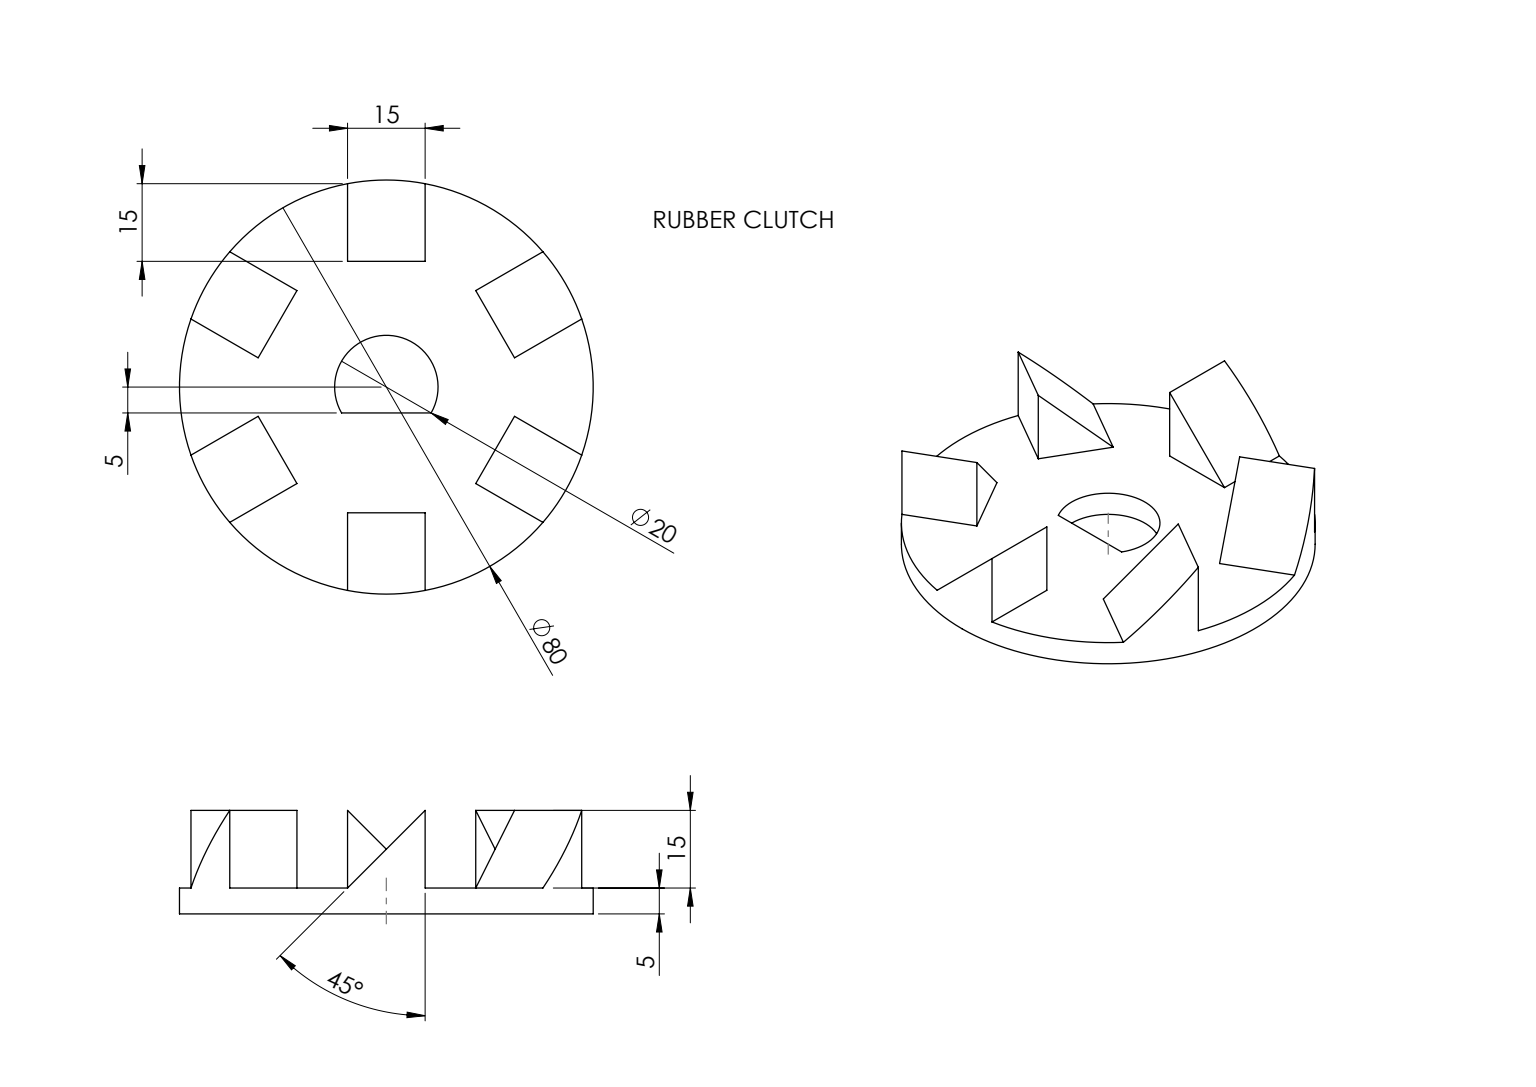
ISO-10303-21;
HEADER;
FILE_DESCRIPTION (('STEP AP214'),
    '1' );
FILE_NAME ('rubber clutch.step',
    '2026-10-09T15:02:13',
    ( '' ),
    ( '' ),
    'SwSTEP 2.0',
    'SolidWorks 2026',
    '' );
FILE_SCHEMA (( 'AUTOMOTIVE_DESIGN' ));
ENDSEC;

DATA;
#35=DIRECTION ( 'NONE',  ( -0.8660254037844327124, 0.000000000000000000, 0.5000000000000102141 ) ) ;
#37=CARTESIAN_POINT ( 'NONE',  ( -24.78626291527390890, 25.00000000000000355, 5.650101528493965297 ) ) ;
#42=CARTESIAN_POINT ( 'NONE',  ( 30.27664397204074476, 25.00000000000000355, 26.14048258526015189 ) ) ;
#92=LINE ( 'NONE', #7754, #12118 ) ;
#146=VECTOR ( 'NONE', #14798, 1000.000000000000000 ) ;
#147=EDGE_CURVE ( 'NONE', #1228, #14186, #15189, .T. ) ;
#226=ORIENTED_EDGE ( 'NONE', *, *, #2314, .T. ) ;
#245=VECTOR ( 'NONE', #10822, 1000.000000000000000 ) ;
#246=ORIENTED_EDGE ( 'NONE', *, *, #11483, .F. ) ;
#251=EDGE_CURVE ( 'NONE', #6737, #5002, #13879, .T. ) ;
#290=LINE ( 'NONE', #6642, #14465 ) ;
#316=SURFACE_SIDE_STYLE ('',( #6586 ) ) ;
#331=VECTOR ( 'NONE', #11777, 1000.000000000000000 ) ;
#372=CARTESIAN_POINT ( 'NONE',  ( -37.77664397204053159, 25.00000000000000355, -13.15010152849376190 ) ) ;
#379=ORIENTED_EDGE ( 'NONE', *, *, #147, .T. ) ;
#392=CARTESIAN_POINT ( 'NONE',  ( -37.77664397204053159, 40.00000000000000711, -13.15010152849376190 ) ) ;
#411=DIRECTION ( 'NONE',  ( -1.000000000000000000, 0.000000000000000000, 2.312964634635742464E-16 ) ) ;
#415=ADVANCED_FACE ( 'NONE', ( #16162 ), #4535, .F. ) ;
#455=EDGE_LOOP ( 'NONE', ( #15919, #7029, #1227 ) ) ;
#484=CARTESIAN_POINT ( 'NONE',  ( 24.78626291527386272, 25.00000000000000355, -5.650101528494135827 ) ) ;
#489=ORIENTED_EDGE ( 'NONE', *, *, #10675, .F. ) ;
#493=DIRECTION ( 'NONE',  ( -0.3535533905932818355, -0.7071067811865463515, -0.6123724356957914727 ) ) ;
#513=ORIENTED_EDGE ( 'NONE', *, *, #11703, .T. ) ;
#524=DIRECTION ( 'NONE',  ( -0.8660254037844399289, 0.000000000000000000, -0.4999999999999976685 ) ) ;
#532=VERTEX_POINT ( 'NONE', #12078 ) ;
#577=EDGE_CURVE ( 'NONE', #11849, #532, #92, .T. ) ;
#585=ORIENTED_EDGE ( 'NONE', *, *, #16374, .T. ) ;
#611=EDGE_LOOP ( 'NONE', ( #10773, #246, #14152, #10214 ) ) ;
#616=DIRECTION ( 'NONE',  ( 0.8660254037844398178, 0.000000000000000000, 0.4999999999999978351 ) ) ;
#641=ORIENTED_EDGE ( 'NONE', *, *, #12919, .T. ) ;
#644=ORIENTED_EDGE ( 'NONE', *, *, #6590, .T. ) ;
#661=STYLED_ITEM ( 'NONE', ( #15532 ), #11759 ) ;
#667=ORIENTED_EDGE ( 'NONE', *, *, #5236, .F. ) ;
#680=VECTOR ( 'NONE', #908, 1000.000000000000000 ) ;
#713=FACE_OUTER_BOUND ( 'NONE', #12733, .T. ) ;
#718=ORIENTED_EDGE ( 'NONE', *, *, #251, .F. ) ;
#758=VERTEX_POINT ( 'NONE', #14387 ) ;
#761=VERTEX_POINT ( 'NONE', #6932 ) ;
#776=MECHANICAL_DESIGN_GEOMETRIC_PRESENTATION_REPRESENTATION('',(#10358),#14324);
#813=LINE ( 'NONE', #10649, #1917 ) ;
#847=FACE_OUTER_BOUND ( 'NONE', #8952, .T. ) ;
#856=AXIS2_PLACEMENT_3D ( 'NONE', #7471, #15025, #3813 ) ;
#858=ORIENTED_EDGE ( 'NONE', *, *, #1166, .T. ) ;
#879=LINE ( 'NONE', #9875, #7578 ) ;
#908=DIRECTION ( 'NONE',  ( 0.5000000000000103251, 0.000000000000000000, 0.8660254037844327124 ) ) ;
#963=EDGE_CURVE ( 'NONE', #14610, #15483, #2393, .T. ) ;
#972=AXIS2_PLACEMENT_3D ( 'NONE', #1664, #10655, #11808 ) ;
#1009=EDGE_CURVE ( 'NONE', #14610, #7079, #9830, .T. ) ;
#1028=ORIENTED_EDGE ( 'NONE', *, *, #8675, .T. ) ;
#1056=CARTESIAN_POINT ( 'NONE',  ( 7.500000000000000000, 40.00000000000000711, 39.29058411375427795 ) ) ;
#1084=CARTESIAN_POINT ( 'NONE',  ( -5.026048470455315886, 27.47395152954465658, 39.76282541253125657 ) ) ;
#1166=EDGE_CURVE ( 'NONE', #13357, #14824, #3055, .T. ) ;
#1181=VERTEX_POINT ( 'NONE', #2335 ) ;
#1202=AXIS2_PLACEMENT_3D ( 'NONE', #5086, #7723, #7477 ) ;
#1210=FACE_OUTER_BOUND ( 'NONE', #4894, .T. ) ;
#1220=DIRECTION ( 'NONE',  ( 0.8660254037844362651, 0.000000000000000000, -0.5000000000000041078 ) ) ;
#1227=ORIENTED_EDGE ( 'NONE', *, *, #9501, .T. ) ;
#1228=VERTEX_POINT ( 'NONE', #484 ) ;
#1231=FACE_OUTER_BOUND ( 'NONE', #5883, .T. ) ;
#1234=( NAMED_UNIT ( * ) SI_UNIT ( $, .STERADIAN. ) SOLID_ANGLE_UNIT ( ) );
#1242=CARTESIAN_POINT ( 'NONE',  ( -36.11321354817274454, 29.97008732934370911, 17.92868204048091840 ) ) ;
#1253=DIRECTION ( 'NONE',  ( 1.000000000000000000, 0.000000000000000000, -2.312964634635742464E-16 ) ) ;
#1282=CIRCLE ( 'NONE', #7664, 40.00000000000000000 ) ;
#1293=DIRECTION ( 'NONE',  ( 0.5000000000000103251, -0.000000000000000000, 0.8660254037844328234 ) ) ;
#1294=CARTESIAN_POINT ( 'NONE',  ( 7.500000000000000000, 25.00000000000000355, 39.29058411375427795 ) ) ;
#1312=COLOUR_RGB ( '', 0.40784314, 0.44705882, 0.49803922) ;
#1317=FACE_OUTER_BOUND ( 'NONE', #13678, .T. ) ;
#1334=EDGE_CURVE ( 'NONE', #13357, #2225, #2828, .T. ) ;
#1374=DIRECTION ( 'NONE',  ( 0.8660254037844327124, 0.000000000000000000, -0.5000000000000102141 ) ) ;
#1386=ORIENTED_EDGE ( 'NONE', *, *, #12039, .T. ) ;
#1399=DIRECTION ( 'NONE',  ( 3.469446951953613696E-16, 0.000000000000000000, 1.000000000000000000 ) ) ;
#1401=AXIS2_PLACEMENT_3D ( 'NONE', #13433, #9616, #10867 ) ;
#1415=ORIENTED_EDGE ( 'NONE', *, *, #13921, .T. ) ;
#1426=CIRCLE ( 'NONE', #12850, 40.00000000000000000 ) ;
#1434=EDGE_CURVE ( 'NONE', #7069, #11084, #1969, .T. ) ;
#1435=UNCERTAINTY_MEASURE_WITH_UNIT (LENGTH_MEASURE( 1.000000000000000082E-05 ), #1651, 'distance_accuracy_value', 'NONE');
#1461=VECTOR ( 'NONE', #16017, 1000.000000000000000 ) ;
#1501=ORIENTED_EDGE ( 'NONE', *, *, #1657, .T. ) ;
#1502=VECTOR ( 'NONE', #1672, 999.9999999999998863 ) ;
#1519=AXIS2_PLACEMENT_3D ( 'NONE', #13845, #1293, #1374 ) ;
#1525=ORIENTED_EDGE ( 'NONE', *, *, #1009, .T. ) ;
#1556=AXIS2_PLACEMENT_3D ( 'NONE', #10146, #14040, #6409 ) ;
#1579=CARTESIAN_POINT ( 'NONE',  ( -17.28626291527383785, 25.00000000000000355, 18.64048258526051427 ) ) ;
#1615=PRODUCT_DEFINITION_SHAPE ( 'NONE', 'NONE',  #14821 ) ;
#1620=ORIENTED_EDGE ( 'NONE', *, *, #4694, .T. ) ;
#1625=EDGE_CURVE ( 'NONE', #3391, #14186, #2782, .T. ) ;
#1651=( LENGTH_UNIT ( ) NAMED_UNIT ( * ) SI_UNIT ( .MILLI., .METRE. ) );
#1657=EDGE_CURVE ( 'NONE', #2087, #5830, #2424, .T. ) ;
#1658=VERTEX_POINT ( 'NONE', #1579 ) ;
#1664=CARTESIAN_POINT ( 'NONE',  ( 0.000000000000000000, 25.00000000000000355, 0.000000000000000000 ) ) ;
#1672=DIRECTION ( 'NONE',  ( -0.8660254037844361541, 0.000000000000000000, 0.5000000000000043299 ) ) ;
#1679=AXIS2_PLACEMENT_3D ( 'NONE', #3745, #10067, #1399 ) ;
#1723=DIRECTION ( 'NONE',  ( 0.000000000000000000, 1.000000000000000000, 0.000000000000000000 ) ) ;
#1812=DIRECTION ( 'NONE',  ( -0.5000000000000041078, 0.000000000000000000, -0.8660254037844363761 ) ) ;
#1824=CARTESIAN_POINT ( 'NONE',  ( -37.77664397204053159, 25.00000000000000355, -13.15010152849376190 ) ) ;
#1843=ORIENTED_EDGE ( 'NONE', *, *, #16366, .F. ) ;
#1848=CARTESIAN_POINT ( 'NONE',  ( -7.500000000000000000, 40.00000000000000711, -39.29058411375427795 ) ) ;
#1851=CARTESIAN_POINT ( 'NONE',  ( 7.500000000000005329, 25.00000000000000355, -24.29058411375428506 ) ) ;
#1861=EDGE_LOOP ( 'NONE', ( #9094, #13992, #14105, #15765 ) ) ;
#1878=ORIENTED_EDGE ( 'NONE', *, *, #3264, .F. ) ;
#1887=DIRECTION ( 'NONE',  ( 0.8660254037844434816, -0.000000000000000000, 0.4999999999999916733 ) ) ;
#1899=FACE_OUTER_BOUND ( 'NONE', #3217, .T. ) ;
#1917=VECTOR ( 'NONE', #11886, 1000.000000000000114 ) ;
#1955=ORIENTED_EDGE ( 'NONE', *, *, #14733, .T. ) ;
#1969=LINE ( 'NONE', #4568, #8682 ) ;
#1971=EDGE_CURVE ( 'NONE', #13357, #6818, #8791, .T. ) ;
#1972=CARTESIAN_POINT ( 'NONE',  ( 0.000000000000000000, 25.00000000000000355, 0.000000000000000000 ) ) ;
#1978=ORIENTED_EDGE ( 'NONE', *, *, #9479, .T. ) ;
#1983=EDGE_LOOP ( 'NONE', ( #585, #8284, #2592, #12178 ) ) ;
#1992=CARTESIAN_POINT ( 'NONE',  ( 37.77664397204061686, 40.00000000000000711, 13.15010152849349900 ) ) ;
#2019=VECTOR ( 'NONE', #16042, 1000.000000000000000 ) ;
#2029=AXIS2_PLACEMENT_3D ( 'NONE', #11411, #2419, #1253 ) ;
#2047=ORIENTED_EDGE ( 'NONE', *, *, #1166, .F. ) ;
#2048=ORIENTED_EDGE ( 'NONE', *, *, #1434, .T. ) ;
#2066=ORIENTED_EDGE ( 'NONE', *, *, #6208, .F. ) ;
#2087=VERTEX_POINT ( 'NONE', #14850 ) ;
#2090=ORIENTED_EDGE ( 'NONE', *, *, #11787, .T. ) ;
#2111=DIRECTION ( 'NONE',  ( 0.000000000000000000, 1.000000000000000000, 0.000000000000000000 ) ) ;
#2135=ADVANCED_FACE ( 'NONE', ( #7219 ), #8534, .F. ) ;
#2158=CARTESIAN_POINT ( 'NONE',  ( 0.000000000000000000, 0.000000000000000000, 0.000000000000000000 ) ) ;
#2172=CARTESIAN_POINT ( 'NONE',  ( -30.27664397204038593, 25.00000000000000355, 26.14048258526057467 ) ) ;
#2173=LINE ( 'NONE', #13488, #9734 ) ;
#2200=VECTOR ( 'NONE', #9579, 1000.000000000000227 ) ;
#2209=CARTESIAN_POINT ( 'NONE',  ( 0.000000000000000000, 20.00000000000000355, 0.000000000000000000 ) ) ;
#2212=LINE ( 'NONE', #15943, #10347 ) ;
#2214=PLANE ( 'NONE',  #15033 ) ;
#2223=EDGE_CURVE ( 'NONE', #6735, #758, #10126, .T. ) ;
#2225=VERTEX_POINT ( 'NONE', #2632 ) ;
#2241=CARTESIAN_POINT ( 'NONE',  ( 37.77664397204061686, 25.00000000000000355, 13.15010152849349900 ) ) ;
#2271=VERTEX_POINT ( 'NONE', #5149 ) ;
#2276=ORIENTED_EDGE ( 'NONE', *, *, #6208, .T. ) ;
#2314=EDGE_CURVE ( 'NONE', #761, #12474, #1282, .T. ) ;
#2329=VECTOR ( 'NONE', #1220, 999.9999999999998863 ) ;
#2335=CARTESIAN_POINT ( 'NONE',  ( 30.27664397204019409, 25.00000000000000355, -26.14048258526078072 ) ) ;
#2340=EDGE_LOOP ( 'NONE', ( #12527, #12705 ) ) ;
#2360=ORIENTED_EDGE ( 'NONE', *, *, #1971, .F. ) ;
#2385=DIRECTION ( 'NONE',  ( 0.000000000000000000, 1.000000000000000000, 0.000000000000000000 ) ) ;
#2393=( BOUNDED_CURVE ( )  B_SPLINE_CURVE ( 3, ( #6008, #10830, #9582, #7252 ),
 .UNSPECIFIED., .F., .F. ) 
 B_SPLINE_CURVE_WITH_KNOTS ( ( 4, 4 ),
 ( 4.523772594209285458, 4.712388980384689674 ),
 .UNSPECIFIED. ) 
 CURVE ( )  GEOMETRIC_REPRESENTATION_ITEM ( )  RATIONAL_B_SPLINE_CURVE ( ( 1.000000000000000000, 0.9970375182503885547, 0.9970375182503885547, 1.000000000000000000 ) ) 
 REPRESENTATION_ITEM ( '' )  );
#2419=DIRECTION ( 'NONE',  ( 2.312964634635742464E-16, -0.000000000000000000, 1.000000000000000000 ) ) ;
#2424=( BOUNDED_CURVE ( )  B_SPLINE_CURVE ( 3, ( #9395, #10571, #4328, #13054 ),
 .UNSPECIFIED., .F., .T. ) 
 B_SPLINE_CURVE_WITH_KNOTS ( ( 4, 4 ),
 ( 4.712388980384689674, 4.901005366560093890 ),
 .UNSPECIFIED. ) 
 CURVE ( )  GEOMETRIC_REPRESENTATION_ITEM ( )  RATIONAL_B_SPLINE_CURVE ( ( 1.000000000000000000, 0.9970375182503885547, 0.9970375182503885547, 1.000000000000000000 ) ) 
 REPRESENTATION_ITEM ( '' )  );
#2436=ORIENTED_EDGE ( 'NONE', *, *, #5698, .F. ) ;
#2439=EDGE_LOOP ( 'NONE', ( #6445, #15228, #12358, #5102, #1525 ) ) ;
#2457=AXIS2_PLACEMENT_3D ( 'NONE', #1972, #13216, #3068 ) ;
#2499=LINE ( 'NONE', #10238, #8412 ) ;
#2516=VERTEX_POINT ( 'NONE', #13471 ) ;
#2517=VECTOR ( 'NONE', #616, 1000.000000000000114 ) ;
#2541=CIRCLE ( 'NONE', #5733, 40.00000000000000000 ) ;
#2561=ADVANCED_FACE ( 'NONE', ( #8981 ), #11314, .F. ) ;
#2571=( LENGTH_UNIT ( ) NAMED_UNIT ( * ) SI_UNIT ( .MILLI., .METRE. ) );
#2592=ORIENTED_EDGE ( 'NONE', *, *, #1625, .F. ) ;
#2632=CARTESIAN_POINT ( 'NONE',  ( -30.27664397204038593, 25.00000000000000355, 26.14048258526057467 ) ) ;
#2657=EDGE_CURVE ( 'NONE', #5002, #2769, #8724, .T. ) ;
#2708=DIRECTION ( 'NONE',  ( -0.3535533905932727872, -0.7071067811865462405, 0.6123724356957966908 ) ) ;
#2724=EDGE_CURVE ( 'NONE', #3391, #5387, #4786, .T. ) ;
#2726=FACE_OUTER_BOUND ( 'NONE', #6080, .T. ) ;
#2747=CARTESIAN_POINT ( 'NONE',  ( -8.660254037844387298, 20.00000000000000355, 5.000000000000000000 ) ) ;
#2765=( BOUNDED_CURVE ( )  B_SPLINE_CURVE ( 3, ( #5034, #10086, #15136, #3763 ),
 .UNSPECIFIED., .F., .F. ) 
 B_SPLINE_CURVE_WITH_KNOTS ( ( 4, 4 ),
 ( 4.523772594209285458, 4.901005366560093002 ),
 .UNSPECIFIED. ) 
 CURVE ( )  GEOMETRIC_REPRESENTATION_ITEM ( )  RATIONAL_B_SPLINE_CURVE ( ( 1.000000000000000000, 0.9881764018959044993, 0.9881764018959044993, 1.000000000000000000 ) ) 
 REPRESENTATION_ITEM ( '' )  );
#2769=VERTEX_POINT ( 'NONE', #15775 ) ;
#2782=LINE ( 'NONE', #11604, #16387 ) ;
#2792=VECTOR ( 'NONE', #7140, 1000.000000000000000 ) ;
#2797=CARTESIAN_POINT ( 'NONE',  ( 24.78626291527397285, 40.00000000000000711, 5.650101528493621572 ) ) ;
#2802=AXIS2_PLACEMENT_3D ( 'NONE', #13583, #2111, #14828 ) ;
#2815=FILL_AREA_STYLE_COLOUR ( '', #1312 ) ;
#2828=LINE ( 'NONE', #14121, #4187 ) ;
#2835=VECTOR ( 'NONE', #5105, 1000.000000000000000 ) ;
#2871=ADVANCED_FACE ( 'NONE', ( #5500 ), #2908, .F. ) ;
#2908=PLANE ( 'NONE',  #12718 ) ;
#2921=CYLINDRICAL_SURFACE ( 'NONE', #972, 40.00000000000000000 ) ;
#2958=DIRECTION ( 'NONE',  ( -0.000000000000000000, -1.000000000000000000, -0.000000000000000000 ) ) ;
#3000=EDGE_CURVE ( 'NONE', #14186, #6058, #2212, .T. ) ;
#3004=LINE ( 'NONE', #9253, #1502 ) ;
#3055=( BOUNDED_CURVE ( )  B_SPLINE_CURVE ( 3, ( #10073, #7734, #1242, #6337 ),
 .UNSPECIFIED., .F., .T. ) 
 B_SPLINE_CURVE_WITH_KNOTS ( ( 4, 4 ),
 ( 4.523772594209285458, 4.901005366560093002 ),
 .UNSPECIFIED. ) 
 CURVE ( )  GEOMETRIC_REPRESENTATION_ITEM ( )  RATIONAL_B_SPLINE_CURVE ( ( 1.000000000000000000, 0.9881764018959044993, 0.9881764018959044993, 1.000000000000000000 ) ) 
 REPRESENTATION_ITEM ( '' )  );
#3068=DIRECTION ( 'NONE',  ( 0.000000000000000000, -0.000000000000000000, 1.000000000000000000 ) ) ;
#3100=ORIENTED_EDGE ( 'NONE', *, *, #6422, .F. ) ;
#3110=EDGE_CURVE ( 'NONE', #9620, #10200, #6470, .T. ) ;
#3135=ORIENTED_EDGE ( 'NONE', *, *, #1334, .F. ) ;
#3140=LINE ( 'NONE', #7970, #6262 ) ;
#3215=ORIENTED_EDGE ( 'NONE', *, *, #6051, .T. ) ;
#3217=EDGE_LOOP ( 'NONE', ( #4738, #5370, #12298, #6596 ) ) ;
#3243=DIRECTION ( 'NONE',  ( 0.3535533905932672916, 0.7071067811865486830, -0.6123724356957968018 ) ) ;
#3264=EDGE_CURVE ( 'NONE', #5374, #758, #10897, .T. ) ;
#3327=DIRECTION ( 'NONE',  ( -0.000000000000000000, -1.000000000000000000, -0.000000000000000000 ) ) ;
#3357=DIRECTION ( 'NONE',  ( 0.8660254037844433705, 0.000000000000000000, 0.4999999999999916178 ) ) ;
#3389=ORIENTED_EDGE ( 'NONE', *, *, #7533, .T. ) ;
#3391=VERTEX_POINT ( 'NONE', #7081 ) ;
#3440=LINE ( 'NONE', #2172, #7521 ) ;
#3445=LINE ( 'NONE', #6028, #16395 ) ;
#3483=DIRECTION ( 'NONE',  ( 0.8660254037844433705, 0.000000000000000000, 0.4999999999999918399 ) ) ;
#3497=EDGE_CURVE ( 'NONE', #14319, #11849, #13789, .T. ) ;
#3540=DIRECTION ( 'NONE',  ( 1.000000000000000000, 0.000000000000000000, 0.000000000000000000 ) ) ;
#3564=CARTESIAN_POINT ( 'NONE',  ( 0.000000000000000000, 25.00000000000000355, 0.000000000000000000 ) ) ;
#3636=MANIFOLD_SOLID_BREP ( 'Cut-Extrude1', #13180 ) ;
#3646=PLANE ( 'NONE',  #1519 ) ;
#3660=ORIENTED_EDGE ( 'NONE', *, *, #7533, .F. ) ;
#3661=ORIENTED_EDGE ( 'NONE', *, *, #9501, .F. ) ;
#3738=ORIENTED_EDGE ( 'NONE', *, *, #9953, .T. ) ;
#3745=CARTESIAN_POINT ( 'NONE',  ( 7.499999999999987566, 40.00000000000000711, -2.602085213965205908E-15 ) ) ;
#3763=CARTESIAN_POINT ( 'NONE',  ( -30.27664397204056712, 25.00000000000000355, -26.14048258526036150 ) ) ;
#3773=DIRECTION ( 'NONE',  ( -0.7071067811865465735, 0.7071067811865484609, 1.635512977795596615E-16 ) ) ;
#3797=CARTESIAN_POINT ( 'NONE',  ( 24.78626291527397285, 25.00000000000000355, 5.650101528493621572 ) ) ;
#3802=CARTESIAN_POINT ( 'NONE',  ( 37.77664397204061686, 40.00000000000000711, 13.15010152849349900 ) ) ;
#3811=AXIS2_PLACEMENT_3D ( 'NONE', #12967, #1812, #6664 ) ;
#3813=DIRECTION ( 'NONE',  ( 0.000000000000000000, 0.000000000000000000, 1.000000000000000000 ) ) ;
#3824=PRESENTATION_STYLE_ASSIGNMENT (( #9228 ) ) ;
#3825=CARTESIAN_POINT ( 'NONE',  ( -7.499999999999998224, 25.00000000000000355, -24.29058411375428150 ) ) ;
#3887=DIRECTION ( 'NONE',  ( 0.000000000000000000, 0.000000000000000000, 1.000000000000000000 ) ) ;
#3907=VECTOR ( 'NONE', #6345, 1000.000000000000000 ) ;
#4028=CARTESIAN_POINT ( 'NONE',  ( -37.77664397204053159, 40.00000000000000711, -13.15010152849376190 ) ) ;
#4067=DIRECTION ( 'NONE',  ( 0.4999999999999978351, 0.000000000000000000, -0.8660254037844399289 ) ) ;
#4069=VECTOR ( 'NONE', #13568, 1000.000000000000114 ) ;
#4077=ORIENTED_EDGE ( 'NONE', *, *, #14561, .T. ) ;
#4084=FACE_OUTER_BOUND ( 'NONE', #12288, .T. ) ;
#4113=ADVANCED_FACE ( 'NONE', ( #1210 ), #10293, .F. ) ;
#4148=PRODUCT ( 'rubber clutch', 'rubber clutch', '', ( #6965 ) ) ;
#4165=FILL_AREA_STYLE ('',( #7895 ) ) ;
#4187=VECTOR ( 'NONE', #10570, 1000.000000000000000 ) ;
#4191=AXIS2_PLACEMENT_3D ( 'NONE', #6061, #13601, #4740 ) ;
#4196=DIRECTION ( 'NONE',  ( -0.8660254037844433705, 0.000000000000000000, -0.4999999999999918399 ) ) ;
#4206=DIRECTION ( 'NONE',  ( -3.469446951953613696E-16, 0.000000000000000000, -1.000000000000000000 ) ) ;
#4231=ORIENTED_EDGE ( 'NONE', *, *, #14339, .T. ) ;
#4236=EDGE_LOOP ( 'NONE', ( #16168, #5571, #11686, #5971 ) ) ;
#4247=( NAMED_UNIT ( * ) PLANE_ANGLE_UNIT ( ) SI_UNIT ( $, .RADIAN. ) );
#4299=LINE ( 'NONE', #14341, #15282 ) ;
#4328=CARTESIAN_POINT ( 'NONE',  ( 5.026048470455315886, 27.47395152954465658, -39.76282541253125657 ) ) ;
#4340=VERTEX_POINT ( 'NONE', #8687 ) ;
#4345=EDGE_CURVE ( 'NONE', #6737, #12652, #6014, .T. ) ;
#4387=EDGE_CURVE ( 'NONE', #12652, #6737, #13752, .T. ) ;
#4418=CARTESIAN_POINT ( 'NONE',  ( 7.499999999999998224, 25.00000000000000355, 24.29058411375428150 ) ) ;
#4535=PLANE ( 'NONE',  #14750 ) ;
#4556=EDGE_LOOP ( 'NONE', ( #15723, #8270, #13295 ) ) ;
#4568=CARTESIAN_POINT ( 'NONE',  ( -24.78626291527393377, 25.00000000000000355, -5.650101528493794767 ) ) ;
#4571=ORIENTED_EDGE ( 'NONE', *, *, #11373, .F. ) ;
#4604=CARTESIAN_POINT ( 'NONE',  ( 0.000000000000000000, 25.00000000000000355, 0.000000000000000000 ) ) ;
#4651=DIRECTION ( 'NONE',  ( -0.000000000000000000, -1.000000000000000000, -0.000000000000000000 ) ) ;
#4694=EDGE_CURVE ( 'NONE', #14169, #2087, #13757, .T. ) ;
#4696=ADVANCED_FACE ( 'NONE', ( #6622 ), #10679, .F. ) ;
#4738=ORIENTED_EDGE ( 'NONE', *, *, #147, .F. ) ;
#4740=DIRECTION ( 'NONE',  ( -1.156482317317871478E-16, 0.000000000000000000, -1.000000000000000000 ) ) ;
#4769=CARTESIAN_POINT ( 'NONE',  ( 30.27664397204019409, 25.00000000000000355, -26.14048258526078072 ) ) ;
#4785=CARTESIAN_POINT ( 'NONE',  ( 3.750000000000036859, 40.00000000000000711, 6.495190528383278483 ) ) ;
#4786=( BOUNDED_CURVE ( )  B_SPLINE_CURVE ( 3, ( #6243, #13954, #12797, #8808 ),
 .UNSPECIFIED., .F., .T. ) 
 B_SPLINE_CURVE_WITH_KNOTS ( ( 4, 4 ),
 ( 4.523772594209285458, 4.901005366560093890 ),
 .UNSPECIFIED. ) 
 CURVE ( )  GEOMETRIC_REPRESENTATION_ITEM ( )  RATIONAL_B_SPLINE_CURVE ( ( 1.000000000000000000, 0.9881764018959044993, 0.9881764018959044993, 1.000000000000000000 ) ) 
 REPRESENTATION_ITEM ( '' )  );
#4793=DIRECTION ( 'NONE',  ( 0.3535533905932685128, -0.7071067811865462405, -0.6123724356957990222 ) ) ;
#4822=LINE ( 'NONE', #12361, #1461 ) ;
#4849=LINE ( 'NONE', #4769, #2200 ) ;
#4856=EDGE_CURVE ( 'NONE', #1228, #5387, #2173, .T. ) ;
#4883=VECTOR ( 'NONE', #6935, 999.9999999999998863 ) ;
#4894=EDGE_LOOP ( 'NONE', ( #8044, #2276, #12130, #7281 ) ) ;
#4897=CARTESIAN_POINT ( 'NONE',  ( -8.660254037844387298, 20.00000000000000355, 5.000000000000000000 ) ) ;
#4922=DIRECTION ( 'NONE',  ( -0.3535533905932715104, 0.7071067811865487940, 0.6123724356957942483 ) ) ;
#5002=VERTEX_POINT ( 'NONE', #9924 ) ;
#5005=ORIENTED_EDGE ( 'NONE', *, *, #6590, .F. ) ;
#5014=PLANE ( 'NONE',  #14232 ) ;
#5028=CARTESIAN_POINT ( 'NONE',  ( 4.898587196589413026E-15, 32.49999999999999289, 40.00000000000000000 ) ) ;
#5034=CARTESIAN_POINT ( 'NONE',  ( -37.77664397204053159, 40.00000000000000711, -13.15010152849376190 ) ) ;
#5053=EDGE_CURVE ( 'NONE', #15026, #14824, #3004, .T. ) ;
#5072=DIRECTION ( 'NONE',  ( -0.8660254037844400399, 0.000000000000000000, -0.4999999999999976685 ) ) ;
#5086=CARTESIAN_POINT ( 'NONE',  ( 0.000000000000000000, 25.00000000000000355, 0.000000000000000000 ) ) ;
#5093=DIRECTION ( 'NONE',  ( -0.8660254037844362651, 0.000000000000000000, 0.5000000000000041078 ) ) ;
#5102=ORIENTED_EDGE ( 'NONE', *, *, #963, .F. ) ;
#5105=DIRECTION ( 'NONE',  ( -0.5000000000000042188, 0.000000000000000000, -0.8660254037844361541 ) ) ;
#5149=CARTESIAN_POINT ( 'NONE',  ( -7.500000000000000000, 25.00000000000000355, 39.29058411375428506 ) ) ;
#5202=ORIENTED_EDGE ( 'NONE', *, *, #12196, .T. ) ;
#5214=EDGE_CURVE ( 'NONE', #2087, #12474, #6854, .T. ) ;
#5236=EDGE_CURVE ( 'NONE', #6058, #1228, #5837, .T. ) ;
#5240=CARTESIAN_POINT ( 'NONE',  ( 7.500000000000000000, 25.00000000000000355, 39.29058411375427795 ) ) ;
#5245=AXIS2_PLACEMENT_3D ( 'NONE', #4604, #9664, #16309 ) ;
#5342=DIRECTION ( 'NONE',  ( -2.312964634635742464E-16, 0.000000000000000000, -1.000000000000000000 ) ) ;
#5353=DIRECTION ( 'NONE',  ( 1.156482317317871478E-16, 0.000000000000000000, 1.000000000000000000 ) ) ;
#5370=ORIENTED_EDGE ( 'NONE', *, *, #4856, .T. ) ;
#5374=VERTEX_POINT ( 'NONE', #2797 ) ;
#5387=VERTEX_POINT ( 'NONE', #7871 ) ;
#5426=EDGE_LOOP ( 'NONE', ( #13925, #3661, #2360, #9220 ) ) ;
#5437=DIRECTION ( 'NONE',  ( -0.4999999999999977796, 0.000000000000000000, 0.8660254037844399289 ) ) ;
#5445=LINE ( 'NONE', #13241, #6201 ) ;
#5481=CIRCLE ( 'NONE', #13419, 40.00000000000000000 ) ;
#5495=VECTOR ( 'NONE', #8882, 1000.000000000000114 ) ;
#5499=DIRECTION ( 'NONE',  ( -0.8660254037844399289, 0.000000000000000000, -0.4999999999999978351 ) ) ;
#5500=FACE_OUTER_BOUND ( 'NONE', #15959, .T. ) ;
#5556=AXIS2_PLACEMENT_3D ( 'NONE', #2209, #7306, #3887 ) ;
#5570=DIRECTION ( 'NONE',  ( 0.8660254037844327124, 0.000000000000000000, -0.5000000000000103251 ) ) ;
#5571=ORIENTED_EDGE ( 'NONE', *, *, #9953, .F. ) ;
#5651=CARTESIAN_POINT ( 'NONE',  ( -24.78626291527393732, 25.00000000000000355, -5.650101528493794767 ) ) ;
#5663=CARTESIAN_POINT ( 'NONE',  ( -3.750000000000069278, 40.00000000000000711, -6.495190528383228745 ) ) ;
#5689=CARTESIAN_POINT ( 'NONE',  ( -5.026048470455357631, 37.52604847045536474, -39.76282541253124947 ) ) ;
#5698=EDGE_CURVE ( 'NONE', #11702, #7069, #12017, .T. ) ;
#5733=AXIS2_PLACEMENT_3D ( 'NONE', #13236, #15644, #15560 ) ;
#5797=PLANE ( 'NONE',  #1401 ) ;
#5830=VERTEX_POINT ( 'NONE', #14744 ) ;
#5837=LINE ( 'NONE', #12306, #680 ) ;
#5843=DIRECTION ( 'NONE',  ( -1.156482317317871478E-16, 0.000000000000000000, -1.000000000000000000 ) ) ;
#5855=DIRECTION ( 'NONE',  ( -0.8660254037844361541, 0.000000000000000000, 0.5000000000000042188 ) ) ;
#5883=EDGE_LOOP ( 'NONE', ( #15156, #12547, #226, #11648, #1501, #3660, #7036, #10674, #10133, #1843, #8414, #15031, #8396 ) ) ;
#5896=DIRECTION ( 'NONE',  ( -0.4999999999999918399, 0.000000000000000000, 0.8660254037844433705 ) ) ;
#5918=LINE ( 'NONE', #10978, #2019 ) ;
#5971=ORIENTED_EDGE ( 'NONE', *, *, #8026, .T. ) ;
#6008=CARTESIAN_POINT ( 'NONE',  ( 7.500000000000000000, 40.00000000000000711, 39.29058411375427795 ) ) ;
#6014=CIRCLE ( 'NONE', #2802, 10.00000000000000000 ) ;
#6015=VECTOR ( 'NONE', #12944, 1000.000000000000000 ) ;
#6024=LINE ( 'NONE', #14976, #4069 ) ;
#6028=CARTESIAN_POINT ( 'NONE',  ( 17.28626291527409720, 25.00000000000000355, 18.64048258526027269 ) ) ;
#6039=ORIENTED_EDGE ( 'NONE', *, *, #4387, .T. ) ;
#6051=EDGE_CURVE ( 'NONE', #11849, #5830, #13327, .T. ) ;
#6058=VERTEX_POINT ( 'NONE', #13088 ) ;
#6061=CARTESIAN_POINT ( 'NONE',  ( -7.500000000000000000, 40.00000000000000711, -39.29058411375427795 ) ) ;
#6072=DIRECTION ( 'NONE',  ( 0.000000000000000000, 1.000000000000000000, 0.000000000000000000 ) ) ;
#6080=EDGE_LOOP ( 'NONE', ( #1978, #718, #10951, #8068 ) ) ;
#6114=DIRECTION ( 'NONE',  ( 0.8660254037844433705, 0.000000000000000000, 0.4999999999999916178 ) ) ;
#6139=CARTESIAN_POINT ( 'NONE',  ( 36.11321354817301454, 35.02991267065631575, 17.92868204048033931 ) ) ;
#6157=ORIENTED_EDGE ( 'NONE', *, *, #5053, .T. ) ;
#6201=VECTOR ( 'NONE', #4196, 1000.000000000000000 ) ;
#6208=EDGE_CURVE ( 'NONE', #11084, #14214, #6873, .T. ) ;
#6215=ORIENTED_EDGE ( 'NONE', *, *, #14733, .F. ) ;
#6239=DIRECTION ( 'NONE',  ( 1.000000000000000000, 0.000000000000000000, -2.312964634635742464E-16 ) ) ;
#6243=CARTESIAN_POINT ( 'NONE',  ( 30.27664397204019409, 40.00000000000000711, -26.14048258526078072 ) ) ;
#6262=VECTOR ( 'NONE', #15444, 1000.000000000000000 ) ;
#6322=ORIENTED_EDGE ( 'NONE', *, *, #12919, .F. ) ;
#6333=CARTESIAN_POINT ( 'NONE',  ( -17.28626291527383785, 40.00000000000000711, 18.64048258526051427 ) ) ;
#6334=EDGE_CURVE ( 'NONE', #10725, #2516, #3445, .T. ) ;
#6337=CARTESIAN_POINT ( 'NONE',  ( -37.77664397204045343, 25.00000000000000355, 13.15010152849403369 ) ) ;
#6345=DIRECTION ( 'NONE',  ( -0.000000000000000000, 1.000000000000000000, -0.000000000000000000 ) ) ;
#6407=DIRECTION ( 'NONE',  ( 0.000000000000000000, 1.000000000000000000, 0.000000000000000000 ) ) ;
#6409=DIRECTION ( 'NONE',  ( 0.000000000000000000, 0.000000000000000000, 1.000000000000000000 ) ) ;
#6410=( NAMED_UNIT ( * ) PLANE_ANGLE_UNIT ( ) SI_UNIT ( $, .RADIAN. ) );
#6422=EDGE_CURVE ( 'NONE', #15026, #6818, #12821, .T. ) ;
#6425=ORIENTED_EDGE ( 'NONE', *, *, #6051, .F. ) ;
#6441=ORIENTED_EDGE ( 'NONE', *, *, #12831, .T. ) ;
#6445=ORIENTED_EDGE ( 'NONE', *, *, #14339, .F. ) ;
#6470=LINE ( 'NONE', #5240, #7943 ) ;
#6586=SURFACE_STYLE_FILL_AREA ( #4165 ) ;
#6590=EDGE_CURVE ( 'NONE', #12474, #761, #2541, .T. ) ;
#6596=ORIENTED_EDGE ( 'NONE', *, *, #1625, .T. ) ;
#6622=FACE_OUTER_BOUND ( 'NONE', #12492, .T. ) ;
#6642=CARTESIAN_POINT ( 'NONE',  ( -24.78626291527393377, 40.00000000000000711, -5.650101528493794767 ) ) ;
#6664=DIRECTION ( 'NONE',  ( -0.8660254037844363761, 0.000000000000000000, 0.5000000000000041078 ) ) ;
#6667=SHAPE_REPRESENTATION_RELATIONSHIP ( 'NONE' , 'NONE' ,  #15095, #11759 ) ;
#6680=ORIENTED_EDGE ( 'NONE', *, *, #16366, .T. ) ;
#6717=LINE ( 'NONE', #15503, #6015 ) ;
#6735=VERTEX_POINT ( 'NONE', #2241 ) ;
#6737=VERTEX_POINT ( 'NONE', #9907 ) ;
#6763=CARTESIAN_POINT ( 'NONE',  ( 0.000000000000000000, 25.00000000000000355, 0.000000000000000000 ) ) ;
#6818=VERTEX_POINT ( 'NONE', #7487 ) ;
#6830=CARTESIAN_POINT ( 'NONE',  ( -7.499999999999998224, 40.00000000000000711, -24.29058411375428150 ) ) ;
#6846=DIRECTION ( 'NONE',  ( 0.8660254037844326014, 0.000000000000000000, -0.5000000000000104361 ) ) ;
#6854=LINE ( 'NONE', #11904, #9997 ) ;
#6873=LINE ( 'NONE', #11924, #14472 ) ;
#6893=DIRECTION ( 'NONE',  ( -0.5000000000000103251, 0.000000000000000000, -0.8660254037844327124 ) ) ;
#6932=CARTESIAN_POINT ( 'NONE',  ( 4.898587196589413026E-15, 20.00000000000000355, 40.00000000000000000 ) ) ;
#6935=DIRECTION ( 'NONE',  ( -0.4999999999999917843, 0.000000000000000000, 0.8660254037844434816 ) ) ;
#6965=PRODUCT_CONTEXT ( 'NONE', #14687, 'mechanical' ) ;
#7002=CARTESIAN_POINT ( 'NONE',  ( -24.78626291527393377, 40.00000000000000711, -5.650101528493794767 ) ) ;
#7029=ORIENTED_EDGE ( 'NONE', *, *, #6422, .T. ) ;
#7036=ORIENTED_EDGE ( 'NONE', *, *, #9462, .F. ) ;
#7044=CARTESIAN_POINT ( 'NONE',  ( 17.28626291527370284, 40.00000000000000711, -18.64048258526063151 ) ) ;
#7069=VERTEX_POINT ( 'NONE', #5651 ) ;
#7079=VERTEX_POINT ( 'NONE', #10568 ) ;
#7081=CARTESIAN_POINT ( 'NONE',  ( 30.27664397204019409, 40.00000000000000711, -26.14048258526078072 ) ) ;
#7118=ORIENTED_EDGE ( 'NONE', *, *, #2223, .T. ) ;
#7140=DIRECTION ( 'NONE',  ( 1.000000000000000000, 0.000000000000000000, 0.000000000000000000 ) ) ;
#7183=PLANE ( 'NONE',  #15199 ) ;
#7219=FACE_OUTER_BOUND ( 'NONE', #611, .T. ) ;
#7221=FACE_OUTER_BOUND ( 'NONE', #4556, .T. ) ;
#7233=ORIENTED_EDGE ( 'NONE', *, *, #9316, .F. ) ;
#7252=CARTESIAN_POINT ( 'NONE',  ( 4.898587196589413026E-15, 32.49999999999999289, 40.00000000000000000 ) ) ;
#7267=DIRECTION ( 'NONE',  ( 0.8660254037844362651, 0.000000000000000000, -0.5000000000000041078 ) ) ;
#7275=VECTOR ( 'NONE', #8643, 1000.000000000000000 ) ;
#7281=ORIENTED_EDGE ( 'NONE', *, *, #15377, .T. ) ;
#7306=DIRECTION ( 'NONE',  ( -0.000000000000000000, 1.000000000000000000, -0.000000000000000000 ) ) ;
#7342=EDGE_LOOP ( 'NONE', ( #9203, #379, #15520 ) ) ;
#7387=CARTESIAN_POINT ( 'NONE',  ( 33.58330087751676984, 29.97008732934371622, 22.31061932476934118 ) ) ;
#7442=( BOUNDED_CURVE ( )  B_SPLINE_CURVE ( 3, ( #3802, #6139, #7387, #42 ),
 .UNSPECIFIED., .F., .F. ) 
 B_SPLINE_CURVE_WITH_KNOTS ( ( 4, 4 ),
 ( 4.523772594209285458, 4.901005366560093002 ),
 .UNSPECIFIED. ) 
 CURVE ( )  GEOMETRIC_REPRESENTATION_ITEM ( )  RATIONAL_B_SPLINE_CURVE ( ( 1.000000000000000000, 0.9881764018959044993, 0.9881764018959044993, 1.000000000000000000 ) ) 
 REPRESENTATION_ITEM ( '' )  );
#7471=CARTESIAN_POINT ( 'NONE',  ( 0.000000000000000000, 25.00000000000000355, 0.000000000000000000 ) ) ;
#7477=DIRECTION ( 'NONE',  ( 0.000000000000000000, 0.000000000000000000, -1.000000000000000000 ) ) ;
#7483=CARTESIAN_POINT ( 'NONE',  ( -7.500000000000005329, 25.00000000000000355, 24.29058411375428506 ) ) ;
#7487=CARTESIAN_POINT ( 'NONE',  ( -17.28626291527383785, 40.00000000000000711, 18.64048258526051427 ) ) ;
#7497=LINE ( 'NONE', #7576, #2835 ) ;
#7521=VECTOR ( 'NONE', #7267, 999.9999999999998863 ) ;
#7533=EDGE_CURVE ( 'NONE', #1181, #5830, #1426, .T. ) ;
#7543=DIRECTION ( 'NONE',  ( 0.000000000000000000, 1.000000000000000000, 0.000000000000000000 ) ) ;
#7576=CARTESIAN_POINT ( 'NONE',  ( -17.28626291527383785, 25.00000000000000355, 18.64048258526051427 ) ) ;
#7578=VECTOR ( 'NONE', #8460, 1000.000000000000000 ) ;
#7623=ORIENTED_EDGE ( 'NONE', *, *, #11598, .T. ) ;
#7664=AXIS2_PLACEMENT_3D ( 'NONE', #13848, #7543, #12613 ) ;
#7723=DIRECTION ( 'NONE',  ( -0.000000000000000000, -1.000000000000000000, -0.000000000000000000 ) ) ;
#7729=PLANE ( 'NONE',  #1679 ) ;
#7734=CARTESIAN_POINT ( 'NONE',  ( -33.58330087751641457, 35.02991267065630154, 22.31061932476987053 ) ) ;
#7754=CARTESIAN_POINT ( 'NONE',  ( -7.499999999999994671, 40.00000000000000711, -24.29058411375428150 ) ) ;
#7801=ORIENTED_EDGE ( 'NONE', *, *, #13221, .T. ) ;
#7804=DIRECTION ( 'NONE',  ( 1.000000000000000000, 0.000000000000000000, 0.000000000000000000 ) ) ;
#7819=ORIENTED_EDGE ( 'NONE', *, *, #13921, .F. ) ;
#7871=CARTESIAN_POINT ( 'NONE',  ( 37.77664397204034685, 25.00000000000000355, -13.15010152849429481 ) ) ;
#7895=FILL_AREA_STYLE_COLOUR ( '', #12889 ) ;
#7943=VECTOR ( 'NONE', #10128, 1000.000000000000000 ) ;
#7960=CARTESIAN_POINT ( 'NONE',  ( -7.500000000000000000, 25.00000000000000355, -39.29058411375427795 ) ) ;
#7964=CARTESIAN_POINT ( 'NONE',  ( 17.28626291527370284, 40.00000000000000711, -18.64048258526062085 ) ) ;
#7970=CARTESIAN_POINT ( 'NONE',  ( 4.898587196589413026E-15, 25.00000000000000355, 40.00000000000000000 ) ) ;
#8026=EDGE_CURVE ( 'NONE', #4340, #11702, #9346, .T. ) ;
#8027=CIRCLE ( 'NONE', #856, 40.00000000000000000 ) ;
#8044=ORIENTED_EDGE ( 'NONE', *, *, #12039, .F. ) ;
#8068=ORIENTED_EDGE ( 'NONE', *, *, #11483, .T. ) ;
#8119=VECTOR ( 'NONE', #3540, 1000.000000000000000 ) ;
#8174=LINE ( 'NONE', #3797, #4883 ) ;
#8182=CARTESIAN_POINT ( 'NONE',  ( 0.000000000000000000, 32.49999999999998579, -40.00000000000000000 ) ) ;
#8206=FACE_OUTER_BOUND ( 'NONE', #7342, .T. ) ;
#8225=FACE_OUTER_BOUND ( 'NONE', #13155, .T. ) ;
#8229=VECTOR ( 'NONE', #6239, 1000.000000000000000 ) ;
#8231=EDGE_LOOP ( 'NONE', ( #6039, #15343 ) ) ;
#8270=ORIENTED_EDGE ( 'NONE', *, *, #10483, .T. ) ;
#8284=ORIENTED_EDGE ( 'NONE', *, *, #3000, .F. ) ;
#8295=CARTESIAN_POINT ( 'NONE',  ( 24.78626291527397285, 40.00000000000000711, 5.650101528493621572 ) ) ;
#8307=ORIENTED_EDGE ( 'NONE', *, *, #1657, .F. ) ;
#8347=VERTEX_POINT ( 'NONE', #12940 ) ;
#8376=LINE ( 'NONE', #16198, #16370 ) ;
#8396=ORIENTED_EDGE ( 'NONE', *, *, #12831, .F. ) ;
#8412=VECTOR ( 'NONE', #5353, 1000.000000000000000 ) ;
#8414=ORIENTED_EDGE ( 'NONE', *, *, #12611, .T. ) ;
#8460=DIRECTION ( 'NONE',  ( -0.000000000000000000, -1.000000000000000000, -0.000000000000000000 ) ) ;
#8471=EDGE_LOOP ( 'NONE', ( #7233, #1028, #7819, #3135, #858, #4571, #15153, #7801, #14636, #16450, #1620, #14149, #644 ) ) ;
#8534=CYLINDRICAL_SURFACE ( 'NONE', #5556, 10.00000000000000000 ) ;
#8536=DIRECTION ( 'NONE',  ( 0.4999999999999916178, 0.000000000000000000, -0.8660254037844433705 ) ) ;
#8560=DIRECTION ( 'NONE',  ( 1.000000000000000000, 0.000000000000000000, 0.000000000000000000 ) ) ;
#8618=DIRECTION ( 'NONE',  ( 0.000000000000000000, 0.000000000000000000, 1.000000000000000000 ) ) ;
#8643=DIRECTION ( 'NONE',  ( -0.000000000000000000, -1.000000000000000000, -0.000000000000000000 ) ) ;
#8674=VECTOR ( 'NONE', #411, 1000.000000000000000 ) ;
#8675=EDGE_CURVE ( 'NONE', #15483, #2271, #13162, .T. ) ;
#8682=VECTOR ( 'NONE', #15780, 1000.000000000000114 ) ;
#8687=CARTESIAN_POINT ( 'NONE',  ( -37.77664397204053159, 40.00000000000000711, -13.15010152849376190 ) ) ;
#8708=DIRECTION ( 'NONE',  ( 3.469446951953613696E-16, 0.000000000000000000, 1.000000000000000000 ) ) ;
#8717=ORIENTED_EDGE ( 'NONE', *, *, #10675, .T. ) ;
#8724=CIRCLE ( 'NONE', #1556, 10.00000000000000000 ) ;
#8783=FACE_OUTER_BOUND ( 'NONE', #1983, .T. ) ;
#8791=LINE ( 'NONE', #13855, #2329 ) ;
#8806=CARTESIAN_POINT ( 'NONE',  ( 0.000000000000000000, 20.00000000000000355, 0.000000000000000000 ) ) ;
#8808=CARTESIAN_POINT ( 'NONE',  ( 37.77664397204034685, 25.00000000000000355, -13.15010152849429481 ) ) ;
#8861=CARTESIAN_POINT ( 'NONE',  ( -7.500000000000000000, 25.00000000000000355, -39.29058411375427795 ) ) ;
#8882=DIRECTION ( 'NONE',  ( -0.3535533905932803922, 0.7071067811865487940, -0.6123724356957891413 ) ) ;
#8884=ORIENTED_EDGE ( 'NONE', *, *, #6334, .F. ) ;
#8888=( NAMED_UNIT ( * ) PLANE_ANGLE_UNIT ( ) SI_UNIT ( $, .RADIAN. ) );
#8952=EDGE_LOOP ( 'NONE', ( #3100, #6157, #2047, #15835 ) ) ;
#8958=CARTESIAN_POINT ( 'NONE',  ( 37.77664397204061686, 25.00000000000000355, 13.15010152849349900 ) ) ;
#8968=ADVANCED_FACE ( 'NONE', ( #2726 ), #15115, .F. ) ;
#8981=FACE_OUTER_BOUND ( 'NONE', #455, .T. ) ;
#9007=AXIS2_PLACEMENT_3D ( 'NONE', #6333, #5093, #13871 ) ;
#9053=ORIENTED_EDGE ( 'NONE', *, *, #3497, .F. ) ;
#9091=VERTEX_POINT ( 'NONE', #10140 ) ;
#9094=ORIENTED_EDGE ( 'NONE', *, *, #10483, .F. ) ;
#9098=DIRECTION ( 'NONE',  ( -0.000000000000000000, -1.000000000000000000, -0.000000000000000000 ) ) ;
#9165=PLANE ( 'NONE',  #14411 ) ;
#9183=CARTESIAN_POINT ( 'NONE',  ( -2.518620260143848100, 35.01862026014384099, -40.00000000000000711 ) ) ;
#9203=ORIENTED_EDGE ( 'NONE', *, *, #5236, .T. ) ;
#9220=ORIENTED_EDGE ( 'NONE', *, *, #1334, .T. ) ;
#9228=SURFACE_STYLE_USAGE ( .BOTH. , #10390 ) ;
#9253=CARTESIAN_POINT ( 'NONE',  ( -24.78626291527390890, 25.00000000000000355, 5.650101528493965297 ) ) ;
#9310=FACE_OUTER_BOUND ( 'NONE', #5426, .T. ) ;
#9316=EDGE_CURVE ( 'NONE', #15483, #761, #3140, .T. ) ;
#9346=LINE ( 'NONE', #4028, #9945 ) ;
#9395=CARTESIAN_POINT ( 'NONE',  ( 0.000000000000000000, 32.49999999999998579, -40.00000000000000000 ) ) ;
#9403=PLANE ( 'NONE',  #13451 ) ;
#9424=AXIS2_PLACEMENT_3D ( 'NONE', #12876, #12546, #7804 ) ;
#9462=EDGE_CURVE ( 'NONE', #3391, #1181, #4822, .T. ) ;
#9479=EDGE_CURVE ( 'NONE', #2769, #5002, #12199, .T. ) ;
#9501=EDGE_CURVE ( 'NONE', #6818, #1658, #879, .T. ) ;
#9547=CARTESIAN_POINT ( 'NONE',  ( 0.000000000000000000, 20.00000000000000355, -40.00000000000000000 ) ) ;
#9575=LINE ( 'NONE', #14619, #11562 ) ;
#9579=DIRECTION ( 'NONE',  ( -0.8660254037844327124, 0.000000000000000000, 0.5000000000000102141 ) ) ;
#9582=CARTESIAN_POINT ( 'NONE',  ( 2.518620260143848100, 35.01862026014384099, 40.00000000000000711 ) ) ;
#9616=DIRECTION ( 'NONE',  ( -1.000000000000000000, 0.000000000000000000, 1.156482317317871478E-16 ) ) ;
#9620=VERTEX_POINT ( 'NONE', #1294 ) ;
#9647=LINE ( 'NONE', #14699, #11835 ) ;
#9664=DIRECTION ( 'NONE',  ( 0.000000000000000000, 1.000000000000000000, 0.000000000000000000 ) ) ;
#9734=VECTOR ( 'NONE', #16157, 1000.000000000000000 ) ;
#9830=LINE ( 'NONE', #12233, #13459 ) ;
#9875=CARTESIAN_POINT ( 'NONE',  ( -17.28626291527383785, 40.00000000000000711, 18.64048258526051427 ) ) ;
#9904=AXIS2_PLACEMENT_3D ( 'NONE', #7044, #5570, #6893 ) ;
#9907=CARTESIAN_POINT ( 'NONE',  ( 8.660254037844387298, 20.00000000000000355, 5.000000000000000000 ) ) ;
#9918=ORIENTED_EDGE ( 'NONE', *, *, #3110, .T. ) ;
#9924=CARTESIAN_POINT ( 'NONE',  ( 8.660254037844387298, 25.00000000000000355, 5.000000000000000000 ) ) ;
#9930=AXIS2_PLACEMENT_3D ( 'NONE', #392, #4067, #5499 ) ;
#9945=VECTOR ( 'NONE', #9098, 1000.000000000000000 ) ;
#9953=EDGE_CURVE ( 'NONE', #8347, #7069, #290, .T. ) ;
#9997=VECTOR ( 'NONE', #14544, 1000.000000000000000 ) ;
#10027=VECTOR ( 'NONE', #4922, 1000.000000000000114 ) ;
#10067=DIRECTION ( 'NONE',  ( 0.7071067811865484609, -0.7071067811865465735, -2.453269466693401579E-16 ) ) ;
#10073=CARTESIAN_POINT ( 'NONE',  ( -30.27664397204038593, 40.00000000000000711, 26.14048258526057467 ) ) ;
#10086=CARTESIAN_POINT ( 'NONE',  ( -36.11321354817288665, 35.02991267065632286, -17.92868204048059155 ) ) ;
#10126=LINE ( 'NONE', #8958, #11643 ) ;
#10128=DIRECTION ( 'NONE',  ( -1.156482317317871478E-16, 0.000000000000000000, -1.000000000000000000 ) ) ;
#10133=ORIENTED_EDGE ( 'NONE', *, *, #12196, .F. ) ;
#10140=CARTESIAN_POINT ( 'NONE',  ( 37.77664397204061686, 40.00000000000000711, 13.15010152849349900 ) ) ;
#10146=CARTESIAN_POINT ( 'NONE',  ( 0.000000000000000000, 25.00000000000000355, 0.000000000000000000 ) ) ;
#10147=( LENGTH_UNIT ( ) NAMED_UNIT ( * ) SI_UNIT ( .MILLI., .METRE. ) );
#10179=ORIENTED_EDGE ( 'NONE', *, *, #11373, .T. ) ;
#10200=VERTEX_POINT ( 'NONE', #14057 ) ;
#10201=ORIENTED_EDGE ( 'NONE', *, *, #15079, .F. ) ;
#10214=ORIENTED_EDGE ( 'NONE', *, *, #251, .T. ) ;
#10238=CARTESIAN_POINT ( 'NONE',  ( -7.500000000000000000, 40.00000000000000711, -39.29058411375427795 ) ) ;
#10273=CIRCLE ( 'NONE', #5245, 40.00000000000000000 ) ;
#10293=PLANE ( 'NONE',  #12094 ) ;
#10301=ORIENTED_EDGE ( 'NONE', *, *, #11787, .F. ) ;
#10314=PLANE ( 'NONE',  #3811 ) ;
#10347=VECTOR ( 'NONE', #4651, 1000.000000000000000 ) ;
#10358=STYLED_ITEM ( 'NONE', ( #3824 ), #3636 ) ;
#10390=SURFACE_SIDE_STYLE ('',( #12792 ) ) ;
#10417=FACE_OUTER_BOUND ( 'NONE', #15056, .T. ) ;
#10433=CARTESIAN_POINT ( 'NONE',  ( -7.499999999999987566, 40.00000000000000711, 2.602085213965205908E-15 ) ) ;
#10479=CARTESIAN_POINT ( 'NONE',  ( -7.500000000000000000, 40.00000000000000711, -39.29058411375427795 ) ) ;
#10483=EDGE_CURVE ( 'NONE', #10725, #5374, #9575, .T. ) ;
#10512=( GEOMETRIC_REPRESENTATION_CONTEXT ( 3 ) GLOBAL_UNCERTAINTY_ASSIGNED_CONTEXT ( ( #14071 ) ) GLOBAL_UNIT_ASSIGNED_CONTEXT ( ( #10147, #6410, #11239 ) ) REPRESENTATION_CONTEXT ( 'NONE', 'WORKASPACE' ) );
#10568=CARTESIAN_POINT ( 'NONE',  ( 7.499999999999998224, 40.00000000000000711, 24.29058411375428150 ) ) ;
#10570=DIRECTION ( 'NONE',  ( -0.000000000000000000, -1.000000000000000000, -0.000000000000000000 ) ) ;
#10571=CARTESIAN_POINT ( 'NONE',  ( 2.518620260143805467, 29.98137973985617677, -40.00000000000000711 ) ) ;
#10578=CARTESIAN_POINT ( 'NONE',  ( 7.500000000000005329, 25.00000000000000355, -24.29058411375428506 ) ) ;
#10584=CARTESIAN_POINT ( 'NONE',  ( 4.898587196589413026E-15, 32.49999999999999289, 40.00000000000000000 ) ) ;
#10636=CARTESIAN_POINT ( 'NONE',  ( 0.000000000000000000, 25.00000000000000355, 0.000000000000000000 ) ) ;
#10649=CARTESIAN_POINT ( 'NONE',  ( 7.499999999999994671, 40.00000000000000711, 24.29058411375428150 ) ) ;
#10655=DIRECTION ( 'NONE',  ( -0.000000000000000000, -1.000000000000000000, -0.000000000000000000 ) ) ;
#10674=ORIENTED_EDGE ( 'NONE', *, *, #2724, .T. ) ;
#10675=EDGE_CURVE ( 'NONE', #532, #14319, #5918, .T. ) ;
#10679=PLANE ( 'NONE',  #11594 ) ;
#10702=VERTEX_POINT ( 'NONE', #7483 ) ;
#10708=DIRECTION ( 'NONE',  ( 0.000000000000000000, 0.000000000000000000, 1.000000000000000000 ) ) ;
#10725=VERTEX_POINT ( 'NONE', #11545 ) ;
#10726=ORIENTED_EDGE ( 'NONE', *, *, #15048, .F. ) ;
#10731=LINE ( 'NONE', #4418, #8674 ) ;
#10773=ORIENTED_EDGE ( 'NONE', *, *, #2657, .T. ) ;
#10780=MECHANICAL_DESIGN_GEOMETRIC_PRESENTATION_REPRESENTATION('',(#661),#13410);
#10822=DIRECTION ( 'NONE',  ( -0.000000000000000000, -1.000000000000000000, -0.000000000000000000 ) ) ;
#10830=CARTESIAN_POINT ( 'NONE',  ( 5.026048470455357631, 37.52604847045536474, 39.76282541253124947 ) ) ;
#10853=ORIENTED_EDGE ( 'NONE', *, *, #11624, .F. ) ;
#10861=ADVANCED_FACE ( 'NONE', ( #16379, #1317 ), #5014, .F. ) ;
#10867=DIRECTION ( 'NONE',  ( 1.156482317317871478E-16, 0.000000000000000000, 1.000000000000000000 ) ) ;
#10897=LINE ( 'NONE', #12396, #245 ) ;
#10951=ORIENTED_EDGE ( 'NONE', *, *, #4387, .F. ) ;
#10978=CARTESIAN_POINT ( 'NONE',  ( -7.499999999999998224, 40.00000000000000711, -24.29058411375428150 ) ) ;
#10989=CARTESIAN_POINT ( 'NONE',  ( 8.660254037844387298, 20.00000000000000355, 5.000000000000000000 ) ) ;
#11054=PRODUCT_DEFINITION_FORMATION_WITH_SPECIFIED_SOURCE ( 'ANY', '', #4148, .NOT_KNOWN. ) ;
#11057=VECTOR ( 'NONE', #14401, 1000.000000000000000 ) ;
#11073=DIRECTION ( 'NONE',  ( 0.000000000000000000, 0.000000000000000000, 1.000000000000000000 ) ) ;
#11084=VERTEX_POINT ( 'NONE', #13994 ) ;
#11193=ORIENTED_EDGE ( 'NONE', *, *, #4856, .F. ) ;
#11239=( NAMED_UNIT ( * ) SI_UNIT ( $, .STERADIAN. ) SOLID_ANGLE_UNIT ( ) );
#11249=EDGE_LOOP ( 'NONE', ( #7118, #1878, #10201, #6680 ) ) ;
#11290=DIRECTION ( 'NONE',  ( -0.8660254037844433705, 0.000000000000000000, -0.4999999999999918399 ) ) ;
#11314=PLANE ( 'NONE',  #9007 ) ;
#11330=CARTESIAN_POINT ( 'NONE',  ( -7.500000000000000000, 25.00000000000000355, 39.29058411375428506 ) ) ;
#11340=CIRCLE ( 'NONE', #12927, 40.00000000000000000 ) ;
#11373=EDGE_CURVE ( 'NONE', #11702, #14824, #10273, .T. ) ;
#11411=CARTESIAN_POINT ( 'NONE',  ( 7.499999999999998224, 40.00000000000000711, 24.29058411375428150 ) ) ;
#11481=PLANE ( 'NONE',  #2029 ) ;
#11483=EDGE_CURVE ( 'NONE', #12652, #2769, #13807, .T. ) ;
#11536=ORIENTED_EDGE ( 'NONE', *, *, #1434, .F. ) ;
#11540=CYLINDRICAL_SURFACE ( 'NONE', #1202, 40.00000000000000000 ) ;
#11545=CARTESIAN_POINT ( 'NONE',  ( 17.28626291527409720, 25.00000000000000355, 18.64048258526027269 ) ) ;
#11559=CARTESIAN_POINT ( 'NONE',  ( -2.518620260143805467, 29.98137973985617677, 40.00000000000000711 ) ) ;
#11562=VECTOR ( 'NONE', #3243, 1000.000000000000114 ) ;
#11594=AXIS2_PLACEMENT_3D ( 'NONE', #10433, #11998, #4206 ) ;
#11598=EDGE_CURVE ( 'NONE', #14169, #532, #2499, .T. ) ;
#11604=CARTESIAN_POINT ( 'NONE',  ( 30.27664397204019409, 40.00000000000000711, -26.14048258526078072 ) ) ;
#11605=ADVANCED_FACE ( 'NONE', ( #4084 ), #11481, .F. ) ;
#11624=EDGE_CURVE ( 'NONE', #1658, #15026, #7497, .T. ) ;
#11643=VECTOR ( 'NONE', #11290, 1000.000000000000000 ) ;
#11648=ORIENTED_EDGE ( 'NONE', *, *, #5214, .F. ) ;
#11686=ORIENTED_EDGE ( 'NONE', *, *, #15377, .F. ) ;
#11702=VERTEX_POINT ( 'NONE', #1824 ) ;
#11703=EDGE_CURVE ( 'NONE', #9620, #2516, #15838, .T. ) ;
#11759=ADVANCED_BREP_SHAPE_REPRESENTATION ( '', ( #3636, #15812 ), #10512 ) ;
#11777=DIRECTION ( 'NONE',  ( 1.156482317317871478E-16, 0.000000000000000000, 1.000000000000000000 ) ) ;
#11779=ADVANCED_FACE ( 'NONE', ( #1899 ), #9403, .F. ) ;
#11787=EDGE_CURVE ( 'NONE', #10200, #10702, #10731, .T. ) ;
#11792=FACE_OUTER_BOUND ( 'NONE', #4236, .T. ) ;
#11808=DIRECTION ( 'NONE',  ( 0.000000000000000000, 0.000000000000000000, -1.000000000000000000 ) ) ;
#11835=VECTOR ( 'NONE', #3327, 1000.000000000000000 ) ;
#11849=VERTEX_POINT ( 'NONE', #10578 ) ;
#11872=ADVANCED_FACE ( 'NONE', ( #14299 ), #2921, .T. ) ;
#11886=DIRECTION ( 'NONE',  ( 0.7071067811865465735, 0.7071067811865484609, -1.635512977795596615E-16 ) ) ;
#11904=CARTESIAN_POINT ( 'NONE',  ( 0.000000000000000000, 25.00000000000000355, -40.00000000000000000 ) ) ;
#11924=CARTESIAN_POINT ( 'NONE',  ( -17.28626291527396930, 25.00000000000000355, -18.64048258526039703 ) ) ;
#11966=ORIENTED_EDGE ( 'NONE', *, *, #2223, .F. ) ;
#11998=DIRECTION ( 'NONE',  ( -0.7071067811865484609, -0.7071067811865465735, 2.453269466693401579E-16 ) ) ;
#12017=LINE ( 'NONE', #372, #2517 ) ;
#12018=SHAPE_DEFINITION_REPRESENTATION ( #1615, #15095 ) ;
#12039=EDGE_CURVE ( 'NONE', #11084, #8347, #14033, .T. ) ;
#12078=CARTESIAN_POINT ( 'NONE',  ( -7.499999999999998224, 40.00000000000000711, -24.29058411375428150 ) ) ;
#12079=ADVANCED_FACE ( 'NONE', ( #1231 ), #11540, .T. ) ;
#12087=ORIENTED_EDGE ( 'NONE', *, *, #577, .T. ) ;
#12094=AXIS2_PLACEMENT_3D ( 'NONE', #16438, #2708, #5072 ) ;
#12118=VECTOR ( 'NONE', #3773, 1000.000000000000114 ) ;
#12124=AXIS2_PLACEMENT_3D ( 'NONE', #6763, #12982, #14450 ) ;
#12130=ORIENTED_EDGE ( 'NONE', *, *, #13221, .F. ) ;
#12178=ORIENTED_EDGE ( 'NONE', *, *, #9462, .T. ) ;
#12182=CARTESIAN_POINT ( 'NONE',  ( -8.660254037844387298, 20.00000000000000355, 5.000000000000000000 ) ) ;
#12196=EDGE_CURVE ( 'NONE', #6735, #5387, #5481, .T. ) ;
#12198=FACE_OUTER_BOUND ( 'NONE', #13521, .T. ) ;
#12199=LINE ( 'NONE', #16192, #2792 ) ;
#12233=CARTESIAN_POINT ( 'NONE',  ( 7.500000000000000000, 40.00000000000000711, 39.29058411375427795 ) ) ;
#12283=CARTESIAN_POINT ( 'NONE',  ( 37.77664397204061686, 40.00000000000000711, 13.15010152849349900 ) ) ;
#12288=EDGE_LOOP ( 'NONE', ( #2090, #4231, #641 ) ) ;
#12298=ORIENTED_EDGE ( 'NONE', *, *, #2724, .F. ) ;
#12306=CARTESIAN_POINT ( 'NONE',  ( 17.28626291527370284, 25.00000000000000355, -18.64048258526063151 ) ) ;
#12358=ORIENTED_EDGE ( 'NONE', *, *, #8675, .F. ) ;
#12361=CARTESIAN_POINT ( 'NONE',  ( 30.27664397204019409, 40.00000000000000711, -26.14048258526078072 ) ) ;
#12396=CARTESIAN_POINT ( 'NONE',  ( 24.78626291527397285, 40.00000000000000711, 5.650101528493621572 ) ) ;
#12416=ADVANCED_FACE ( 'NONE', ( #12198 ), #16107, .F. ) ;
#12474=VERTEX_POINT ( 'NONE', #9547 ) ;
#12492=EDGE_LOOP ( 'NONE', ( #13244, #3215, #8307, #13665, #7623 ) ) ;
#12527=ORIENTED_EDGE ( 'NONE', *, *, #2657, .F. ) ;
#12543=ORIENTED_EDGE ( 'NONE', *, *, #11598, .F. ) ;
#12546=DIRECTION ( 'NONE',  ( -0.000000000000000000, 0.000000000000000000, 1.000000000000000000 ) ) ;
#12547=ORIENTED_EDGE ( 'NONE', *, *, #9316, .T. ) ;
#12611=EDGE_CURVE ( 'NONE', #9091, #2516, #7442, .T. ) ;
#12613=DIRECTION ( 'NONE',  ( 0.000000000000000000, 0.000000000000000000, 1.000000000000000000 ) ) ;
#12623=ADVANCED_FACE ( 'NONE', ( #8783 ), #3646, .F. ) ;
#12652=VERTEX_POINT ( 'NONE', #4897 ) ;
#12705=ORIENTED_EDGE ( 'NONE', *, *, #9479, .F. ) ;
#12716=FILL_AREA_STYLE ('',( #2815 ) ) ;
#12718=AXIS2_PLACEMENT_3D ( 'NONE', #6830, #5342, #14522 ) ;
#12733=EDGE_LOOP ( 'NONE', ( #9918, #6322, #16033, #6441 ) ) ;
#12781=CARTESIAN_POINT ( 'NONE',  ( 0.000000000000000000, 25.00000000000000355, 0.000000000000000000 ) ) ;
#12792=SURFACE_STYLE_FILL_AREA ( #12716 ) ;
#12797=CARTESIAN_POINT ( 'NONE',  ( 36.11321354817260953, 29.97008732934370201, -17.92868204048114222 ) ) ;
#12821=LINE ( 'NONE', #13980, #14765 ) ;
#12831=EDGE_CURVE ( 'NONE', #14610, #9620, #6717, .T. ) ;
#12850=AXIS2_PLACEMENT_3D ( 'NONE', #12781, #6072, #8618 ) ;
#12876=CARTESIAN_POINT ( 'NONE',  ( -8.660254037844387298, 20.00000000000000355, 5.000000000000000000 ) ) ;
#12889=COLOUR_RGB ( '', 0.40784314, 0.44705882, 0.49803922) ;
#12919=EDGE_CURVE ( 'NONE', #7079, #10200, #4299, .T. ) ;
#12927=AXIS2_PLACEMENT_3D ( 'NONE', #3564, #2385, #13689 ) ;
#12940=CARTESIAN_POINT ( 'NONE',  ( -24.78626291527393377, 40.00000000000000711, -5.650101528493794767 ) ) ;
#12944=DIRECTION ( 'NONE',  ( -0.000000000000000000, -1.000000000000000000, -0.000000000000000000 ) ) ;
#12967=CARTESIAN_POINT ( 'NONE',  ( -30.27664397204038593, 40.00000000000000711, 26.14048258526057467 ) ) ;
#12977=CARTESIAN_POINT ( 'NONE',  ( -30.27664397204056712, 25.00000000000000355, -26.14048258526036150 ) ) ;
#12982=DIRECTION ( 'NONE',  ( 0.000000000000000000, 1.000000000000000000, 0.000000000000000000 ) ) ;
#13050=SURFACE_STYLE_USAGE ( .BOTH. , #316 ) ;
#13054=CARTESIAN_POINT ( 'NONE',  ( 7.500000000000000000, 25.00000000000000355, -39.29058411375427795 ) ) ;
#13056=ORIENTED_EDGE ( 'NONE', *, *, #5053, .F. ) ;
#13088=CARTESIAN_POINT ( 'NONE',  ( 17.28626291527369929, 25.00000000000000355, -18.64048258526063151 ) ) ;
#13122=PLANE ( 'NONE',  #9930 ) ;
#13155=EDGE_LOOP ( 'NONE', ( #11193, #667, #16325, #3389, #6425, #9053, #6215, #4077, #2066, #11536, #2436, #10179, #13056, #10853, #15654, #1415, #15112, #10301, #13319, #513, #8884, #10726, #11966, #5202 ) ) ;
#13162=( BOUNDED_CURVE ( )  B_SPLINE_CURVE ( 3, ( #5028, #11559, #1084, #11330 ),
 .UNSPECIFIED., .F., .F. ) 
 B_SPLINE_CURVE_WITH_KNOTS ( ( 4, 4 ),
 ( 4.712388980384689674, 4.901005366560093890 ),
 .UNSPECIFIED. ) 
 CURVE ( )  GEOMETRIC_REPRESENTATION_ITEM ( )  RATIONAL_B_SPLINE_CURVE ( ( 1.000000000000000000, 0.9970375182503885547, 0.9970375182503885547, 1.000000000000000000 ) ) 
 REPRESENTATION_ITEM ( '' )  );
#13180=CLOSED_SHELL ( 'NONE', ( #12079, #11872, #14357, #10861, #12416, #2871, #4696, #16117, #16345, #16071, #2561, #14865, #11605, #13973, #16172, #12623, #14820, #4113, #15286, #15987, #415, #11779, #2135, #8968 ) ) ;
#13200=ORIENTED_EDGE ( 'NONE', *, *, #3497, .T. ) ;
#13216=DIRECTION ( 'NONE',  ( 0.000000000000000000, 1.000000000000000000, 0.000000000000000000 ) ) ;
#13221=EDGE_CURVE ( 'NONE', #4340, #14214, #2765, .T. ) ;
#13236=CARTESIAN_POINT ( 'NONE',  ( 0.000000000000000000, 20.00000000000000355, 0.000000000000000000 ) ) ;
#13241=CARTESIAN_POINT ( 'NONE',  ( 37.77664397204061686, 40.00000000000000711, 13.15010152849349900 ) ) ;
#13244=ORIENTED_EDGE ( 'NONE', *, *, #577, .F. ) ;
#13274=CARTESIAN_POINT ( 'NONE',  ( -37.77664397204045343, 25.00000000000000355, 13.15010152849403369 ) ) ;
#13295=ORIENTED_EDGE ( 'NONE', *, *, #3264, .T. ) ;
#13319=ORIENTED_EDGE ( 'NONE', *, *, #3110, .F. ) ;
#13327=LINE ( 'NONE', #1851, #11057 ) ;
#13357=VERTEX_POINT ( 'NONE', #15711 ) ;
#13363=PLANE ( 'NONE',  #15208 ) ;
#13410=( GEOMETRIC_REPRESENTATION_CONTEXT ( 3 ) GLOBAL_UNCERTAINTY_ASSIGNED_CONTEXT ( ( #1435 ) ) GLOBAL_UNIT_ASSIGNED_CONTEXT ( ( #1651, #4247, #15622 ) ) REPRESENTATION_CONTEXT ( 'NONE', 'WORKASPACE' ) );
#13419=AXIS2_PLACEMENT_3D ( 'NONE', #10636, #1723, #10708 ) ;
#13433=CARTESIAN_POINT ( 'NONE',  ( 7.500000000000000000, 40.00000000000000711, 39.29058411375427795 ) ) ;
#13451=AXIS2_PLACEMENT_3D ( 'NONE', #5663, #493, #6846 ) ;
#13452=FACE_OUTER_BOUND ( 'NONE', #11249, .T. ) ;
#13459=VECTOR ( 'NONE', #5843, 1000.000000000000000 ) ;
#13471=CARTESIAN_POINT ( 'NONE',  ( 30.27664397204074476, 25.00000000000000355, 26.14048258526015189 ) ) ;
#13488=CARTESIAN_POINT ( 'NONE',  ( 24.78626291527386272, 25.00000000000000355, -5.650101528494135827 ) ) ;
#13521=EDGE_LOOP ( 'NONE', ( #1955, #489, #12543, #15574 ) ) ;
#13561=EDGE_CURVE ( 'NONE', #14169, #15028, #9647, .T. ) ;
#13568=DIRECTION ( 'NONE',  ( 0.8660254037844398178, 0.000000000000000000, 0.4999999999999978351 ) ) ;
#13583=CARTESIAN_POINT ( 'NONE',  ( 0.000000000000000000, 20.00000000000000355, 0.000000000000000000 ) ) ;
#13601=DIRECTION ( 'NONE',  ( 1.000000000000000000, 0.000000000000000000, -1.156482317317871478E-16 ) ) ;
#13655=CARTESIAN_POINT ( 'NONE',  ( 3.749999999999932943, 40.00000000000000711, -6.495190528383318451 ) ) ;
#13665=ORIENTED_EDGE ( 'NONE', *, *, #4694, .F. ) ;
#13678=EDGE_LOOP ( 'NONE', ( #5005, #14371 ) ) ;
#13689=DIRECTION ( 'NONE',  ( 0.000000000000000000, 0.000000000000000000, 1.000000000000000000 ) ) ;
#13752=LINE ( 'NONE', #12182, #8119 ) ;
#13757=( BOUNDED_CURVE ( )  B_SPLINE_CURVE ( 3, ( #1848, #5689, #9183, #8182 ),
 .UNSPECIFIED., .F., .F. ) 
 B_SPLINE_CURVE_WITH_KNOTS ( ( 4, 4 ),
 ( 4.523772594209285458, 4.712388980384689674 ),
 .UNSPECIFIED. ) 
 CURVE ( )  GEOMETRIC_REPRESENTATION_ITEM ( )  RATIONAL_B_SPLINE_CURVE ( ( 1.000000000000000000, 0.9970375182503885547, 0.9970375182503885547, 1.000000000000000000 ) ) 
 REPRESENTATION_ITEM ( '' )  );
#13789=LINE ( 'NONE', #3825, #8229 ) ;
#13807=LINE ( 'NONE', #2747, #3907 ) ;
#13845=CARTESIAN_POINT ( 'NONE',  ( 30.27664397204019409, 40.00000000000000711, -26.14048258526078072 ) ) ;
#13848=CARTESIAN_POINT ( 'NONE',  ( 0.000000000000000000, 20.00000000000000355, 0.000000000000000000 ) ) ;
#13855=CARTESIAN_POINT ( 'NONE',  ( -30.27664397204038593, 40.00000000000000711, 26.14048258526057467 ) ) ;
#13871=DIRECTION ( 'NONE',  ( 0.5000000000000041078, 0.000000000000000000, 0.8660254037844362651 ) ) ;
#13879=LINE ( 'NONE', #10989, #146 ) ;
#13914=EDGE_CURVE ( 'NONE', #10702, #2271, #8376, .T. ) ;
#13921=EDGE_CURVE ( 'NONE', #2225, #2271, #11340, .T. ) ;
#13925=ORIENTED_EDGE ( 'NONE', *, *, #15396, .T. ) ;
#13954=CARTESIAN_POINT ( 'NONE',  ( 33.58330087751625825, 35.02991267065631575, -22.31061932477009080 ) ) ;
#13973=ADVANCED_FACE ( 'NONE', ( #13452 ), #2214, .F. ) ;
#13980=CARTESIAN_POINT ( 'NONE',  ( -17.28626291527383430, 40.00000000000000711, 18.64048258526052848 ) ) ;
#13992=ORIENTED_EDGE ( 'NONE', *, *, #6334, .T. ) ;
#13994=CARTESIAN_POINT ( 'NONE',  ( -17.28626291527396930, 25.00000000000000355, -18.64048258526039703 ) ) ;
#14033=LINE ( 'NONE', #16284, #10027 ) ;
#14040=DIRECTION ( 'NONE',  ( 0.000000000000000000, 1.000000000000000000, 0.000000000000000000 ) ) ;
#14046=CARTESIAN_POINT ( 'NONE',  ( 17.28626291527370284, 40.00000000000000711, -18.64048258526063151 ) ) ;
#14057=CARTESIAN_POINT ( 'NONE',  ( 7.499999999999998224, 25.00000000000000355, 24.29058411375428150 ) ) ;
#14070=APPLICATION_CONTEXT ( 'automotive_design' ) ;
#14071=UNCERTAINTY_MEASURE_WITH_UNIT (LENGTH_MEASURE( 1.000000000000000082E-05 ), #10147, 'distance_accuracy_value', 'NONE');
#14105=ORIENTED_EDGE ( 'NONE', *, *, #12611, .F. ) ;
#14121=CARTESIAN_POINT ( 'NONE',  ( -30.27664397204038593, 40.00000000000000711, 26.14048258526057467 ) ) ;
#14149=ORIENTED_EDGE ( 'NONE', *, *, #5214, .T. ) ;
#14152=ORIENTED_EDGE ( 'NONE', *, *, #4345, .F. ) ;
#14169=VERTEX_POINT ( 'NONE', #10479 ) ;
#14186=VERTEX_POINT ( 'NONE', #14046 ) ;
#14214=VERTEX_POINT ( 'NONE', #12977 ) ;
#14232=AXIS2_PLACEMENT_3D ( 'NONE', #8806, #6407, #15280 ) ;
#14236=PRODUCT_DEFINITION_CONTEXT ( 'detailed design', #14070, 'design' ) ;
#14299=FACE_OUTER_BOUND ( 'NONE', #8471, .T. ) ;
#14319=VERTEX_POINT ( 'NONE', #16028 ) ;
#14324=( GEOMETRIC_REPRESENTATION_CONTEXT ( 3 ) GLOBAL_UNCERTAINTY_ASSIGNED_CONTEXT ( ( #15405 ) ) GLOBAL_UNIT_ASSIGNED_CONTEXT ( ( #2571, #8888, #1234 ) ) REPRESENTATION_CONTEXT ( 'NONE', 'WORKASPACE' ) );
#14339=EDGE_CURVE ( 'NONE', #10702, #7079, #813, .T. ) ;
#14341=CARTESIAN_POINT ( 'NONE',  ( 7.499999999999998224, 40.00000000000000711, 24.29058411375428150 ) ) ;
#14357=ADVANCED_FACE ( 'NONE', ( #15702, #8225 ), #14443, .T. ) ;
#14371=ORIENTED_EDGE ( 'NONE', *, *, #2314, .F. ) ;
#14387=CARTESIAN_POINT ( 'NONE',  ( 24.78626291527397285, 25.00000000000000355, 5.650101528493621572 ) ) ;
#14401=DIRECTION ( 'NONE',  ( -3.469446951953613696E-16, 0.000000000000000000, -1.000000000000000000 ) ) ;
#14411=AXIS2_PLACEMENT_3D ( 'NONE', #7002, #15716, #5437 ) ;
#14443=PLANE ( 'NONE',  #2457 ) ;
#14450=DIRECTION ( 'NONE',  ( 0.000000000000000000, 0.000000000000000000, 1.000000000000000000 ) ) ;
#14465=VECTOR ( 'NONE', #15675, 1000.000000000000000 ) ;
#14472=VECTOR ( 'NONE', #524, 1000.000000000000114 ) ;
#14509=PLANE ( 'NONE',  #9904 ) ;
#14522=DIRECTION ( 'NONE',  ( -1.000000000000000000, 0.000000000000000000, 2.312964634635742464E-16 ) ) ;
#14544=DIRECTION ( 'NONE',  ( -0.000000000000000000, -1.000000000000000000, -0.000000000000000000 ) ) ;
#14561=EDGE_CURVE ( 'NONE', #15028, #14214, #8027, .T. ) ;
#14610=VERTEX_POINT ( 'NONE', #1056 ) ;
#14619=CARTESIAN_POINT ( 'NONE',  ( 24.78626291527397285, 40.00000000000000711, 5.650101528493618908 ) ) ;
#14636=ORIENTED_EDGE ( 'NONE', *, *, #14561, .F. ) ;
#14639=DIRECTION ( 'NONE',  ( 0.3535533905932773391, -0.7071067811865463515, 0.6123724356957938042 ) ) ;
#14687=APPLICATION_CONTEXT ( 'automotive_design' ) ;
#14699=CARTESIAN_POINT ( 'NONE',  ( -7.500000000000000000, 40.00000000000000711, -39.29058411375427795 ) ) ;
#14733=EDGE_CURVE ( 'NONE', #15028, #14319, #15514, .T. ) ;
#14744=CARTESIAN_POINT ( 'NONE',  ( 7.500000000000000000, 25.00000000000000355, -39.29058411375427795 ) ) ;
#14750=AXIS2_PLACEMENT_3D ( 'NONE', #13655, #4793, #6114 ) ;
#14765=VECTOR ( 'NONE', #16318, 1000.000000000000114 ) ;
#14798=DIRECTION ( 'NONE',  ( -0.000000000000000000, 1.000000000000000000, -0.000000000000000000 ) ) ;
#14820=ADVANCED_FACE ( 'NONE', ( #8206 ), #14509, .F. ) ;
#14821=PRODUCT_DEFINITION ( 'UNKNOWN', '', #11054, #14236 ) ;
#14824=VERTEX_POINT ( 'NONE', #13274 ) ;
#14828=DIRECTION ( 'NONE',  ( 0.000000000000000000, 0.000000000000000000, 1.000000000000000000 ) ) ;
#14850=CARTESIAN_POINT ( 'NONE',  ( 0.000000000000000000, 32.49999999999998579, -40.00000000000000000 ) ) ;
#14865=ADVANCED_FACE ( 'NONE', ( #713 ), #5797, .F. ) ;
#14976=CARTESIAN_POINT ( 'NONE',  ( -37.77664397204053159, 40.00000000000000711, -13.15010152849376190 ) ) ;
#15025=DIRECTION ( 'NONE',  ( 0.000000000000000000, 1.000000000000000000, 0.000000000000000000 ) ) ;
#15026=VERTEX_POINT ( 'NONE', #37 ) ;
#15028=VERTEX_POINT ( 'NONE', #8861 ) ;
#15031=ORIENTED_EDGE ( 'NONE', *, *, #11703, .F. ) ;
#15033=AXIS2_PLACEMENT_3D ( 'NONE', #12283, #5896, #3483 ) ;
#15048=EDGE_CURVE ( 'NONE', #758, #10725, #8174, .T. ) ;
#15056=EDGE_LOOP ( 'NONE', ( #2048, #1386, #3738 ) ) ;
#15079=EDGE_CURVE ( 'NONE', #9091, #5374, #5445, .T. ) ;
#15095=SHAPE_REPRESENTATION ( 'rubber clutch', ( #15812 ), #10512 ) ;
#15112=ORIENTED_EDGE ( 'NONE', *, *, #13914, .F. ) ;
#15115=PLANE ( 'NONE',  #9424 ) ;
#15136=CARTESIAN_POINT ( 'NONE',  ( -33.58330087751660642, 29.97008732934372333, -22.31061932476956855 ) ) ;
#15153=ORIENTED_EDGE ( 'NONE', *, *, #8026, .F. ) ;
#15156=ORIENTED_EDGE ( 'NONE', *, *, #963, .T. ) ;
#15189=LINE ( 'NONE', #7964, #5495 ) ;
#15199=AXIS2_PLACEMENT_3D ( 'NONE', #4785, #14639, #5855 ) ;
#15208=AXIS2_PLACEMENT_3D ( 'NONE', #8295, #1887, #8536 ) ;
#15228=ORIENTED_EDGE ( 'NONE', *, *, #13914, .T. ) ;
#15280=DIRECTION ( 'NONE',  ( 0.000000000000000000, -0.000000000000000000, 1.000000000000000000 ) ) ;
#15282=VECTOR ( 'NONE', #2958, 1000.000000000000000 ) ;
#15283=FACE_OUTER_BOUND ( 'NONE', #2439, .T. ) ;
#15286=ADVANCED_FACE ( 'NONE', ( #847 ), #7183, .F. ) ;
#15343=ORIENTED_EDGE ( 'NONE', *, *, #4345, .T. ) ;
#15377=EDGE_CURVE ( 'NONE', #4340, #8347, #6024, .T. ) ;
#15396=EDGE_CURVE ( 'NONE', #2225, #1658, #3440, .T. ) ;
#15405=UNCERTAINTY_MEASURE_WITH_UNIT (LENGTH_MEASURE( 1.000000000000000082E-05 ), #2571, 'distance_accuracy_value', 'NONE');
#15444=DIRECTION ( 'NONE',  ( -0.000000000000000000, -1.000000000000000000, -0.000000000000000000 ) ) ;
#15483=VERTEX_POINT ( 'NONE', #10584 ) ;
#15503=CARTESIAN_POINT ( 'NONE',  ( 7.500000000000000000, 40.00000000000000711, 39.29058411375427795 ) ) ;
#15514=LINE ( 'NONE', #7960, #331 ) ;
#15520=ORIENTED_EDGE ( 'NONE', *, *, #3000, .T. ) ;
#15532=PRESENTATION_STYLE_ASSIGNMENT (( #13050 ) ) ;
#15560=DIRECTION ( 'NONE',  ( 0.000000000000000000, 0.000000000000000000, 1.000000000000000000 ) ) ;
#15574=ORIENTED_EDGE ( 'NONE', *, *, #13561, .T. ) ;
#15622=( NAMED_UNIT ( * ) SI_UNIT ( $, .STERADIAN. ) SOLID_ANGLE_UNIT ( ) );
#15644=DIRECTION ( 'NONE',  ( 0.000000000000000000, 1.000000000000000000, 0.000000000000000000 ) ) ;
#15654=ORIENTED_EDGE ( 'NONE', *, *, #15396, .F. ) ;
#15675=DIRECTION ( 'NONE',  ( -0.000000000000000000, -1.000000000000000000, -0.000000000000000000 ) ) ;
#15702=FACE_BOUND ( 'NONE', #2340, .T. ) ;
#15711=CARTESIAN_POINT ( 'NONE',  ( -30.27664397204038593, 40.00000000000000711, 26.14048258526057467 ) ) ;
#15716=DIRECTION ( 'NONE',  ( -0.8660254037844399289, 0.000000000000000000, -0.4999999999999977796 ) ) ;
#15723=ORIENTED_EDGE ( 'NONE', *, *, #15048, .T. ) ;
#15765=ORIENTED_EDGE ( 'NONE', *, *, #15079, .T. ) ;
#15775=CARTESIAN_POINT ( 'NONE',  ( -8.660254037844387298, 25.00000000000000355, 5.000000000000000000 ) ) ;
#15780=DIRECTION ( 'NONE',  ( 0.4999999999999977240, 0.000000000000000000, -0.8660254037844398178 ) ) ;
#15812=AXIS2_PLACEMENT_3D ( 'NONE', #2158, #11073, #8560 ) ;
#15835=ORIENTED_EDGE ( 'NONE', *, *, #1971, .T. ) ;
#15838=CIRCLE ( 'NONE', #12124, 40.00000000000000000 ) ;
#15890=LINE ( 'NONE', #1992, #7275 ) ;
#15919=ORIENTED_EDGE ( 'NONE', *, *, #11624, .T. ) ;
#15943=CARTESIAN_POINT ( 'NONE',  ( 17.28626291527370284, 40.00000000000000711, -18.64048258526063151 ) ) ;
#15959=EDGE_LOOP ( 'NONE', ( #13200, #12087, #8717 ) ) ;
#15987=ADVANCED_FACE ( 'NONE', ( #15283 ), #7729, .F. ) ;
#16017=DIRECTION ( 'NONE',  ( -0.000000000000000000, -1.000000000000000000, -0.000000000000000000 ) ) ;
#16028=CARTESIAN_POINT ( 'NONE',  ( -7.499999999999998224, 25.00000000000000355, -24.29058411375428150 ) ) ;
#16033=ORIENTED_EDGE ( 'NONE', *, *, #1009, .F. ) ;
#16042=DIRECTION ( 'NONE',  ( -0.000000000000000000, -1.000000000000000000, -0.000000000000000000 ) ) ;
#16071=ADVANCED_FACE ( 'NONE', ( #9310 ), #10314, .F. ) ;
#16107=PLANE ( 'NONE',  #4191 ) ;
#16117=ADVANCED_FACE ( 'NONE', ( #11792 ), #13122, .F. ) ;
#16157=DIRECTION ( 'NONE',  ( 0.8660254037844326014, 0.000000000000000000, -0.5000000000000104361 ) ) ;
#16162=FACE_OUTER_BOUND ( 'NONE', #1861, .T. ) ;
#16168=ORIENTED_EDGE ( 'NONE', *, *, #5698, .T. ) ;
#16172=ADVANCED_FACE ( 'NONE', ( #7221 ), #13363, .F. ) ;
#16192=CARTESIAN_POINT ( 'NONE',  ( -8.660254037844387298, 25.00000000000000355, 5.000000000000000000 ) ) ;
#16198=CARTESIAN_POINT ( 'NONE',  ( -7.500000000000005329, 25.00000000000000355, 24.29058411375428506 ) ) ;
#16284=CARTESIAN_POINT ( 'NONE',  ( -24.78626291527393022, 40.00000000000000711, -5.650101528493793879 ) ) ;
#16309=DIRECTION ( 'NONE',  ( 0.000000000000000000, 0.000000000000000000, 1.000000000000000000 ) ) ;
#16318=DIRECTION ( 'NONE',  ( 0.3535533905932762289, 0.7071067811865484609, 0.6123724356957919168 ) ) ;
#16325=ORIENTED_EDGE ( 'NONE', *, *, #16374, .F. ) ;
#16345=ADVANCED_FACE ( 'NONE', ( #10417 ), #9165, .F. ) ;
#16366=EDGE_CURVE ( 'NONE', #9091, #6735, #15890, .T. ) ;
#16370=VECTOR ( 'NONE', #8708, 1000.000000000000000 ) ;
#16374=EDGE_CURVE ( 'NONE', #1181, #6058, #4849, .T. ) ;
#16379=FACE_BOUND ( 'NONE', #8231, .T. ) ;
#16387=VECTOR ( 'NONE', #35, 1000.000000000000227 ) ;
#16395=VECTOR ( 'NONE', #3357, 1000.000000000000114 ) ;
#16438=CARTESIAN_POINT ( 'NONE',  ( -3.749999999999977351, 40.00000000000000711, 6.495190528383290918 ) ) ;
#16450=ORIENTED_EDGE ( 'NONE', *, *, #13561, .F. ) ;
ENDSEC;
END-ISO-10303-21;
